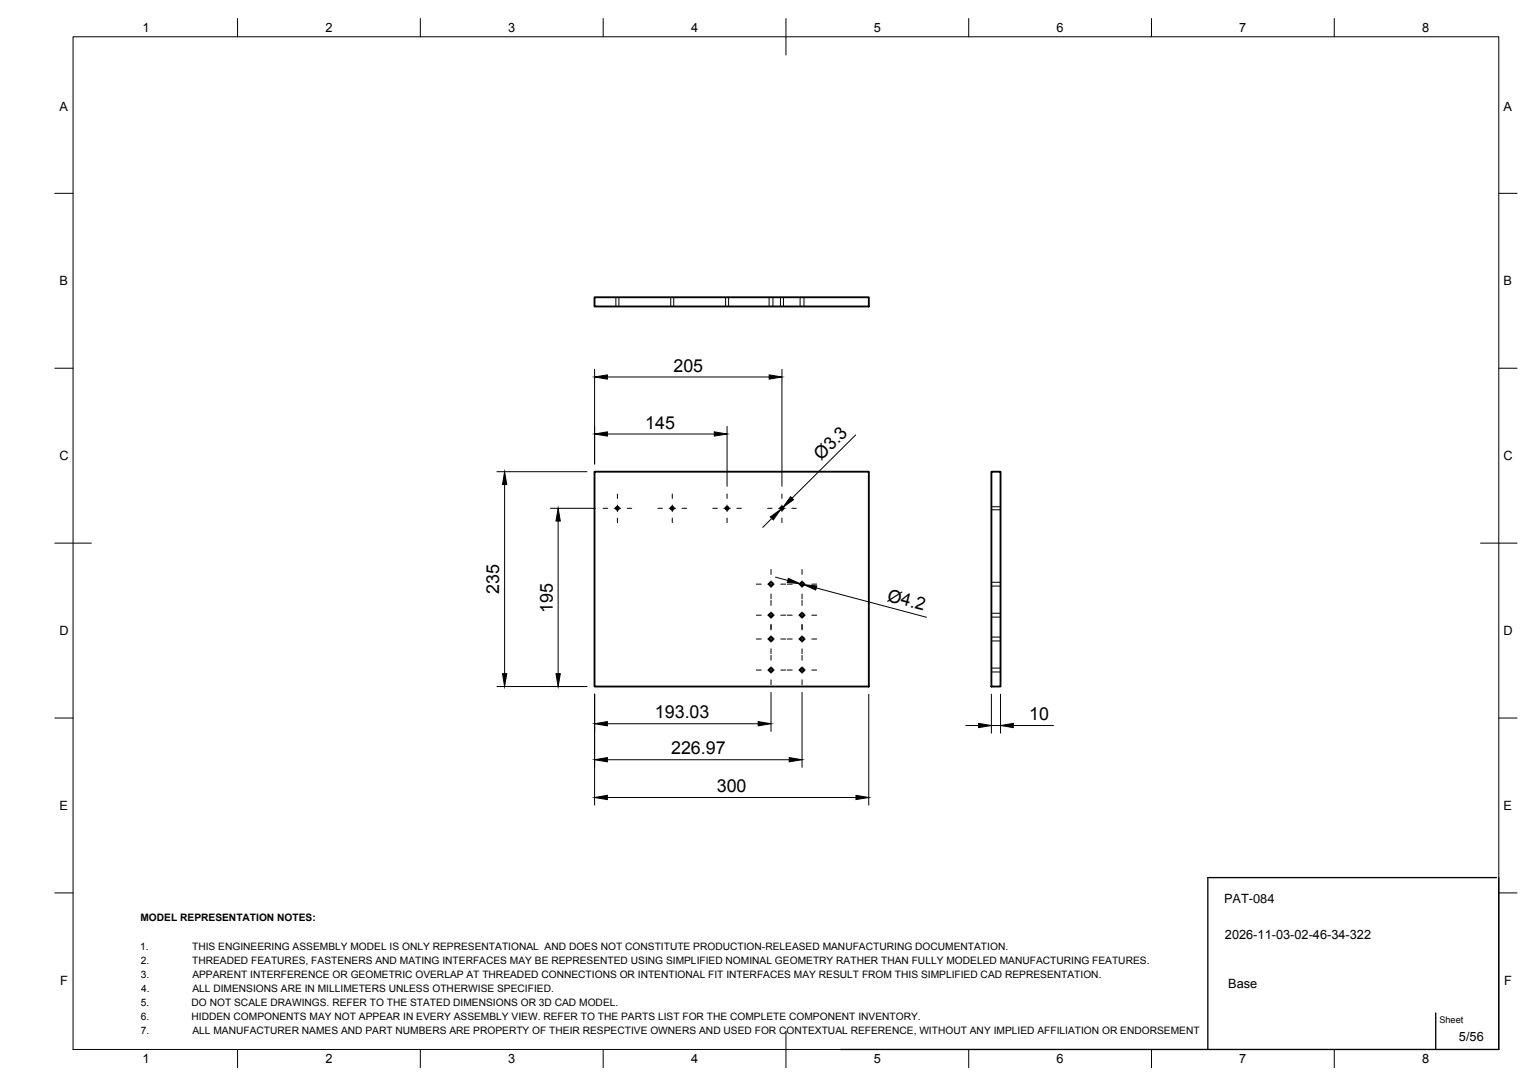
ISO-10303-21;
HEADER;
/* Generated by software containing ST-Developer
 * from STEP Tools, Inc. (www.steptools.com) 
 */

FILE_DESCRIPTION(
/* description */ ('Quick-return (Whitworth) mechanism'),
/* implementation_level */ '2;1');

FILE_NAME(
/* name */ 'Base.step',
/* time_stamp */ '2026-10-28T03:25:57-07:00',
/* author */ (''),
/* organization */ (''),
/* preprocessor_version */ 'ST-DEVELOPER v20.2',
/* originating_system */ 'Autodesk Translation Framework v15.17.0.0',
/* authorisation */ '');

FILE_SCHEMA (('AUTOMOTIVE_DESIGN { 1 0 10303 214 3 1 1 }'));
ENDSEC;

DATA;
#10=MECHANICAL_DESIGN_GEOMETRIC_PRESENTATION_REPRESENTATION('',(#490),#14878);
#402=SHAPE_REPRESENTATION_RELATIONSHIP('SRR','None',#15070,#446);
#446=ADVANCED_BREP_SHAPE_REPRESENTATION('',(#542),#14827);
#490=STYLED_ITEM('',(#15385),#542);
#542=MANIFOLD_SOLID_BREP('Body1',#7844);
#591=FACE_BOUND('',#1530,.T.);
#592=FACE_BOUND('',#1531,.T.);
#593=FACE_BOUND('',#1532,.T.);
#594=FACE_BOUND('',#1533,.T.);
#595=FACE_BOUND('',#1534,.T.);
#596=FACE_BOUND('',#1535,.T.);
#597=FACE_BOUND('',#1536,.T.);
#598=FACE_BOUND('',#1537,.T.);
#599=FACE_BOUND('',#1538,.T.);
#600=FACE_BOUND('',#1539,.T.);
#601=FACE_BOUND('',#1540,.T.);
#602=FACE_BOUND('',#1541,.T.);
#603=FACE_BOUND('',#1543,.T.);
#604=FACE_BOUND('',#1544,.T.);
#605=FACE_BOUND('',#1545,.T.);
#606=FACE_BOUND('',#1546,.T.);
#607=FACE_BOUND('',#1547,.T.);
#608=FACE_BOUND('',#1548,.T.);
#609=FACE_BOUND('',#1549,.T.);
#610=FACE_BOUND('',#1550,.T.);
#611=FACE_BOUND('',#1551,.T.);
#612=FACE_BOUND('',#1552,.T.);
#613=FACE_BOUND('',#1553,.T.);
#614=FACE_BOUND('',#1554,.T.);
#782=PLANE('',#8423);
#783=PLANE('',#8424);
#784=PLANE('',#8425);
#785=PLANE('',#8426);
#786=PLANE('',#8427);
#787=PLANE('',#8428);
#1047=FACE_OUTER_BOUND('',#1513,.T.);
#1048=FACE_OUTER_BOUND('',#1514,.T.);
#1049=FACE_OUTER_BOUND('',#1515,.T.);
#1050=FACE_OUTER_BOUND('',#1516,.T.);
#1051=FACE_OUTER_BOUND('',#1517,.T.);
#1052=FACE_OUTER_BOUND('',#1518,.T.);
#1053=FACE_OUTER_BOUND('',#1519,.T.);
#1054=FACE_OUTER_BOUND('',#1520,.T.);
#1055=FACE_OUTER_BOUND('',#1521,.T.);
#1056=FACE_OUTER_BOUND('',#1522,.T.);
#1057=FACE_OUTER_BOUND('',#1523,.T.);
#1058=FACE_OUTER_BOUND('',#1524,.T.);
#1059=FACE_OUTER_BOUND('',#1525,.T.);
#1060=FACE_OUTER_BOUND('',#1526,.T.);
#1061=FACE_OUTER_BOUND('',#1527,.T.);
#1062=FACE_OUTER_BOUND('',#1528,.T.);
#1063=FACE_OUTER_BOUND('',#1529,.T.);
#1064=FACE_OUTER_BOUND('',#1542,.T.);
#1513=EDGE_LOOP('',(#5262,#5263,#5264,#5265));
#1514=EDGE_LOOP('',(#5266,#5267,#5268,#5269));
#1515=EDGE_LOOP('',(#5270,#5271,#5272,#5273));
#1516=EDGE_LOOP('',(#5274,#5275,#5276,#5277));
#1517=EDGE_LOOP('',(#5278,#5279,#5280,#5281));
#1518=EDGE_LOOP('',(#5282,#5283,#5284,#5285));
#1519=EDGE_LOOP('',(#5286,#5287,#5288,#5289));
#1520=EDGE_LOOP('',(#5290,#5291,#5292,#5293));
#1521=EDGE_LOOP('',(#5294,#5295,#5296,#5297));
#1522=EDGE_LOOP('',(#5298,#5299,#5300,#5301));
#1523=EDGE_LOOP('',(#5302,#5303,#5304,#5305));
#1524=EDGE_LOOP('',(#5306,#5307,#5308,#5309));
#1525=EDGE_LOOP('',(#5310,#5311,#5312,#5313));
#1526=EDGE_LOOP('',(#5314,#5315,#5316,#5317));
#1527=EDGE_LOOP('',(#5318,#5319,#5320,#5321));
#1528=EDGE_LOOP('',(#5322,#5323,#5324,#5325));
#1529=EDGE_LOOP('',(#5326,#5327,#5328,#5329));
#1530=EDGE_LOOP('',(#5330));
#1531=EDGE_LOOP('',(#5331));
#1532=EDGE_LOOP('',(#5332));
#1533=EDGE_LOOP('',(#5333));
#1534=EDGE_LOOP('',(#5334));
#1535=EDGE_LOOP('',(#5335));
#1536=EDGE_LOOP('',(#5336));
#1537=EDGE_LOOP('',(#5337));
#1538=EDGE_LOOP('',(#5338));
#1539=EDGE_LOOP('',(#5339));
#1540=EDGE_LOOP('',(#5340));
#1541=EDGE_LOOP('',(#5341));
#1542=EDGE_LOOP('',(#5342,#5343,#5344,#5345));
#1543=EDGE_LOOP('',(#5346));
#1544=EDGE_LOOP('',(#5347));
#1545=EDGE_LOOP('',(#5348));
#1546=EDGE_LOOP('',(#5349));
#1547=EDGE_LOOP('',(#5350));
#1548=EDGE_LOOP('',(#5351));
#1549=EDGE_LOOP('',(#5352));
#1550=EDGE_LOOP('',(#5353));
#1551=EDGE_LOOP('',(#5354));
#1552=EDGE_LOOP('',(#5355));
#1553=EDGE_LOOP('',(#5356));
#1554=EDGE_LOOP('',(#5357));
#2170=LINE('',#11953,#2693);
#2171=LINE('',#11959,#2694);
#2172=LINE('',#11965,#2695);
#2173=LINE('',#11971,#2696);
#2174=LINE('',#11977,#2697);
#2175=LINE('',#11983,#2698);
#2176=LINE('',#11989,#2699);
#2177=LINE('',#11995,#2700);
#2178=LINE('',#12001,#2701);
#2179=LINE('',#12007,#2702);
#2180=LINE('',#12013,#2703);
#2181=LINE('',#12019,#2704);
#2182=LINE('',#12024,#2705);
#2183=LINE('',#12026,#2706);
#2184=LINE('',#12028,#2707);
#2185=LINE('',#12029,#2708);
#2186=LINE('',#12032,#2709);
#2187=LINE('',#12034,#2710);
#2188=LINE('',#12035,#2711);
#2189=LINE('',#12038,#2712);
#2190=LINE('',#12040,#2713);
#2191=LINE('',#12041,#2714);
#2192=LINE('',#12043,#2715);
#2193=LINE('',#12044,#2716);
#2693=VECTOR('',#9407,0.21);
#2694=VECTOR('',#9414,0.21);
#2695=VECTOR('',#9421,0.21);
#2696=VECTOR('',#9428,0.21);
#2697=VECTOR('',#9435,0.21);
#2698=VECTOR('',#9442,0.21);
#2699=VECTOR('',#9449,0.21);
#2700=VECTOR('',#9456,0.21);
#2701=VECTOR('',#9463,0.164999999999999);
#2702=VECTOR('',#9470,0.164999999999999);
#2703=VECTOR('',#9477,0.165);
#2704=VECTOR('',#9484,0.165);
#2705=VECTOR('',#9489,1.);
#2706=VECTOR('',#9490,1.);
#2707=VECTOR('',#9491,1.);
#2708=VECTOR('',#9492,1.);
#2709=VECTOR('',#9495,1.);
#2710=VECTOR('',#9496,1.);
#2711=VECTOR('',#9497,1.);
#2712=VECTOR('',#9500,1.);
#2713=VECTOR('',#9501,1.);
#2714=VECTOR('',#9502,1.);
#2715=VECTOR('',#9505,1.);
#2716=VECTOR('',#9506,1.);
#3216=CIRCLE('',#8388,0.21);
#3217=CIRCLE('',#8389,0.21);
#3218=CIRCLE('',#8391,0.21);
#3219=CIRCLE('',#8392,0.21);
#3220=CIRCLE('',#8394,0.21);
#3221=CIRCLE('',#8395,0.21);
#3222=CIRCLE('',#8397,0.21);
#3223=CIRCLE('',#8398,0.21);
#3224=CIRCLE('',#8400,0.21);
#3225=CIRCLE('',#8401,0.21);
#3226=CIRCLE('',#8403,0.21);
#3227=CIRCLE('',#8404,0.21);
#3228=CIRCLE('',#8406,0.21);
#3229=CIRCLE('',#8407,0.21);
#3230=CIRCLE('',#8409,0.21);
#3231=CIRCLE('',#8410,0.21);
#3232=CIRCLE('',#8412,0.164999999999999);
#3233=CIRCLE('',#8413,0.164999999999999);
#3234=CIRCLE('',#8415,0.164999999999999);
#3235=CIRCLE('',#8416,0.164999999999999);
#3236=CIRCLE('',#8418,0.165);
#3237=CIRCLE('',#8419,0.165);
#3238=CIRCLE('',#8421,0.165);
#3239=CIRCLE('',#8422,0.165);
#3631=VERTEX_POINT('',#11950);
#3632=VERTEX_POINT('',#11952);
#3633=VERTEX_POINT('',#11956);
#3634=VERTEX_POINT('',#11958);
#3635=VERTEX_POINT('',#11962);
#3636=VERTEX_POINT('',#11964);
#3637=VERTEX_POINT('',#11968);
#3638=VERTEX_POINT('',#11970);
#3639=VERTEX_POINT('',#11974);
#3640=VERTEX_POINT('',#11976);
#3641=VERTEX_POINT('',#11980);
#3642=VERTEX_POINT('',#11982);
#3643=VERTEX_POINT('',#11986);
#3644=VERTEX_POINT('',#11988);
#3645=VERTEX_POINT('',#11992);
#3646=VERTEX_POINT('',#11994);
#3647=VERTEX_POINT('',#11998);
#3648=VERTEX_POINT('',#12000);
#3649=VERTEX_POINT('',#12004);
#3650=VERTEX_POINT('',#12006);
#3651=VERTEX_POINT('',#12010);
#3652=VERTEX_POINT('',#12012);
#3653=VERTEX_POINT('',#12016);
#3654=VERTEX_POINT('',#12018);
#3655=VERTEX_POINT('',#12022);
#3656=VERTEX_POINT('',#12023);
#3657=VERTEX_POINT('',#12025);
#3658=VERTEX_POINT('',#12027);
#3659=VERTEX_POINT('',#12031);
#3660=VERTEX_POINT('',#12033);
#3661=VERTEX_POINT('',#12037);
#3662=VERTEX_POINT('',#12039);
#4288=EDGE_CURVE('',#3631,#3631,#3216,.T.);
#4289=EDGE_CURVE('',#3631,#3632,#2170,.T.);
#4290=EDGE_CURVE('',#3632,#3632,#3217,.T.);
#4291=EDGE_CURVE('',#3633,#3633,#3218,.T.);
#4292=EDGE_CURVE('',#3633,#3634,#2171,.T.);
#4293=EDGE_CURVE('',#3634,#3634,#3219,.T.);
#4294=EDGE_CURVE('',#3635,#3635,#3220,.T.);
#4295=EDGE_CURVE('',#3635,#3636,#2172,.T.);
#4296=EDGE_CURVE('',#3636,#3636,#3221,.T.);
#4297=EDGE_CURVE('',#3637,#3637,#3222,.T.);
#4298=EDGE_CURVE('',#3637,#3638,#2173,.T.);
#4299=EDGE_CURVE('',#3638,#3638,#3223,.T.);
#4300=EDGE_CURVE('',#3639,#3639,#3224,.T.);
#4301=EDGE_CURVE('',#3639,#3640,#2174,.T.);
#4302=EDGE_CURVE('',#3640,#3640,#3225,.T.);
#4303=EDGE_CURVE('',#3641,#3641,#3226,.T.);
#4304=EDGE_CURVE('',#3641,#3642,#2175,.T.);
#4305=EDGE_CURVE('',#3642,#3642,#3227,.T.);
#4306=EDGE_CURVE('',#3643,#3643,#3228,.T.);
#4307=EDGE_CURVE('',#3643,#3644,#2176,.T.);
#4308=EDGE_CURVE('',#3644,#3644,#3229,.T.);
#4309=EDGE_CURVE('',#3645,#3645,#3230,.T.);
#4310=EDGE_CURVE('',#3645,#3646,#2177,.T.);
#4311=EDGE_CURVE('',#3646,#3646,#3231,.T.);
#4312=EDGE_CURVE('',#3647,#3647,#3232,.T.);
#4313=EDGE_CURVE('',#3647,#3648,#2178,.T.);
#4314=EDGE_CURVE('',#3648,#3648,#3233,.T.);
#4315=EDGE_CURVE('',#3649,#3649,#3234,.T.);
#4316=EDGE_CURVE('',#3649,#3650,#2179,.T.);
#4317=EDGE_CURVE('',#3650,#3650,#3235,.T.);
#4318=EDGE_CURVE('',#3651,#3651,#3236,.T.);
#4319=EDGE_CURVE('',#3651,#3652,#2180,.T.);
#4320=EDGE_CURVE('',#3652,#3652,#3237,.T.);
#4321=EDGE_CURVE('',#3653,#3653,#3238,.T.);
#4322=EDGE_CURVE('',#3653,#3654,#2181,.T.);
#4323=EDGE_CURVE('',#3654,#3654,#3239,.T.);
#4324=EDGE_CURVE('',#3655,#3656,#2182,.T.);
#4325=EDGE_CURVE('',#3656,#3657,#2183,.T.);
#4326=EDGE_CURVE('',#3658,#3657,#2184,.T.);
#4327=EDGE_CURVE('',#3655,#3658,#2185,.T.);
#4328=EDGE_CURVE('',#3659,#3655,#2186,.T.);
#4329=EDGE_CURVE('',#3660,#3658,#2187,.T.);
#4330=EDGE_CURVE('',#3659,#3660,#2188,.T.);
#4331=EDGE_CURVE('',#3661,#3659,#2189,.T.);
#4332=EDGE_CURVE('',#3662,#3660,#2190,.T.);
#4333=EDGE_CURVE('',#3661,#3662,#2191,.T.);
#4334=EDGE_CURVE('',#3656,#3661,#2192,.T.);
#4335=EDGE_CURVE('',#3657,#3662,#2193,.T.);
#5262=ORIENTED_EDGE('',*,*,#4288,.F.);
#5263=ORIENTED_EDGE('',*,*,#4289,.T.);
#5264=ORIENTED_EDGE('',*,*,#4290,.F.);
#5265=ORIENTED_EDGE('',*,*,#4289,.F.);
#5266=ORIENTED_EDGE('',*,*,#4291,.F.);
#5267=ORIENTED_EDGE('',*,*,#4292,.T.);
#5268=ORIENTED_EDGE('',*,*,#4293,.F.);
#5269=ORIENTED_EDGE('',*,*,#4292,.F.);
#5270=ORIENTED_EDGE('',*,*,#4294,.F.);
#5271=ORIENTED_EDGE('',*,*,#4295,.T.);
#5272=ORIENTED_EDGE('',*,*,#4296,.F.);
#5273=ORIENTED_EDGE('',*,*,#4295,.F.);
#5274=ORIENTED_EDGE('',*,*,#4297,.F.);
#5275=ORIENTED_EDGE('',*,*,#4298,.T.);
#5276=ORIENTED_EDGE('',*,*,#4299,.F.);
#5277=ORIENTED_EDGE('',*,*,#4298,.F.);
#5278=ORIENTED_EDGE('',*,*,#4300,.F.);
#5279=ORIENTED_EDGE('',*,*,#4301,.T.);
#5280=ORIENTED_EDGE('',*,*,#4302,.F.);
#5281=ORIENTED_EDGE('',*,*,#4301,.F.);
#5282=ORIENTED_EDGE('',*,*,#4303,.F.);
#5283=ORIENTED_EDGE('',*,*,#4304,.T.);
#5284=ORIENTED_EDGE('',*,*,#4305,.F.);
#5285=ORIENTED_EDGE('',*,*,#4304,.F.);
#5286=ORIENTED_EDGE('',*,*,#4306,.F.);
#5287=ORIENTED_EDGE('',*,*,#4307,.T.);
#5288=ORIENTED_EDGE('',*,*,#4308,.F.);
#5289=ORIENTED_EDGE('',*,*,#4307,.F.);
#5290=ORIENTED_EDGE('',*,*,#4309,.F.);
#5291=ORIENTED_EDGE('',*,*,#4310,.T.);
#5292=ORIENTED_EDGE('',*,*,#4311,.F.);
#5293=ORIENTED_EDGE('',*,*,#4310,.F.);
#5294=ORIENTED_EDGE('',*,*,#4312,.F.);
#5295=ORIENTED_EDGE('',*,*,#4313,.T.);
#5296=ORIENTED_EDGE('',*,*,#4314,.F.);
#5297=ORIENTED_EDGE('',*,*,#4313,.F.);
#5298=ORIENTED_EDGE('',*,*,#4315,.F.);
#5299=ORIENTED_EDGE('',*,*,#4316,.T.);
#5300=ORIENTED_EDGE('',*,*,#4317,.F.);
#5301=ORIENTED_EDGE('',*,*,#4316,.F.);
#5302=ORIENTED_EDGE('',*,*,#4318,.F.);
#5303=ORIENTED_EDGE('',*,*,#4319,.T.);
#5304=ORIENTED_EDGE('',*,*,#4320,.F.);
#5305=ORIENTED_EDGE('',*,*,#4319,.F.);
#5306=ORIENTED_EDGE('',*,*,#4321,.F.);
#5307=ORIENTED_EDGE('',*,*,#4322,.T.);
#5308=ORIENTED_EDGE('',*,*,#4323,.F.);
#5309=ORIENTED_EDGE('',*,*,#4322,.F.);
#5310=ORIENTED_EDGE('',*,*,#4324,.T.);
#5311=ORIENTED_EDGE('',*,*,#4325,.T.);
#5312=ORIENTED_EDGE('',*,*,#4326,.F.);
#5313=ORIENTED_EDGE('',*,*,#4327,.F.);
#5314=ORIENTED_EDGE('',*,*,#4328,.T.);
#5315=ORIENTED_EDGE('',*,*,#4327,.T.);
#5316=ORIENTED_EDGE('',*,*,#4329,.F.);
#5317=ORIENTED_EDGE('',*,*,#4330,.F.);
#5318=ORIENTED_EDGE('',*,*,#4331,.T.);
#5319=ORIENTED_EDGE('',*,*,#4330,.T.);
#5320=ORIENTED_EDGE('',*,*,#4332,.F.);
#5321=ORIENTED_EDGE('',*,*,#4333,.F.);
#5322=ORIENTED_EDGE('',*,*,#4334,.T.);
#5323=ORIENTED_EDGE('',*,*,#4333,.T.);
#5324=ORIENTED_EDGE('',*,*,#4335,.F.);
#5325=ORIENTED_EDGE('',*,*,#4325,.F.);
#5326=ORIENTED_EDGE('',*,*,#4335,.T.);
#5327=ORIENTED_EDGE('',*,*,#4332,.T.);
#5328=ORIENTED_EDGE('',*,*,#4329,.T.);
#5329=ORIENTED_EDGE('',*,*,#4326,.T.);
#5330=ORIENTED_EDGE('',*,*,#4302,.T.);
#5331=ORIENTED_EDGE('',*,*,#4305,.T.);
#5332=ORIENTED_EDGE('',*,*,#4308,.T.);
#5333=ORIENTED_EDGE('',*,*,#4311,.T.);
#5334=ORIENTED_EDGE('',*,*,#4314,.T.);
#5335=ORIENTED_EDGE('',*,*,#4317,.T.);
#5336=ORIENTED_EDGE('',*,*,#4320,.T.);
#5337=ORIENTED_EDGE('',*,*,#4323,.T.);
#5338=ORIENTED_EDGE('',*,*,#4299,.T.);
#5339=ORIENTED_EDGE('',*,*,#4296,.T.);
#5340=ORIENTED_EDGE('',*,*,#4293,.T.);
#5341=ORIENTED_EDGE('',*,*,#4290,.T.);
#5342=ORIENTED_EDGE('',*,*,#4334,.F.);
#5343=ORIENTED_EDGE('',*,*,#4324,.F.);
#5344=ORIENTED_EDGE('',*,*,#4328,.F.);
#5345=ORIENTED_EDGE('',*,*,#4331,.F.);
#5346=ORIENTED_EDGE('',*,*,#4300,.T.);
#5347=ORIENTED_EDGE('',*,*,#4303,.T.);
#5348=ORIENTED_EDGE('',*,*,#4306,.T.);
#5349=ORIENTED_EDGE('',*,*,#4309,.T.);
#5350=ORIENTED_EDGE('',*,*,#4312,.T.);
#5351=ORIENTED_EDGE('',*,*,#4315,.T.);
#5352=ORIENTED_EDGE('',*,*,#4318,.T.);
#5353=ORIENTED_EDGE('',*,*,#4321,.T.);
#5354=ORIENTED_EDGE('',*,*,#4297,.T.);
#5355=ORIENTED_EDGE('',*,*,#4294,.T.);
#5356=ORIENTED_EDGE('',*,*,#4291,.T.);
#5357=ORIENTED_EDGE('',*,*,#4288,.T.);
#7210=CYLINDRICAL_SURFACE('',#8387,0.21);
#7211=CYLINDRICAL_SURFACE('',#8390,0.21);
#7212=CYLINDRICAL_SURFACE('',#8393,0.21);
#7213=CYLINDRICAL_SURFACE('',#8396,0.21);
#7214=CYLINDRICAL_SURFACE('',#8399,0.21);
#7215=CYLINDRICAL_SURFACE('',#8402,0.21);
#7216=CYLINDRICAL_SURFACE('',#8405,0.21);
#7217=CYLINDRICAL_SURFACE('',#8408,0.21);
#7218=CYLINDRICAL_SURFACE('',#8411,0.164999999999999);
#7219=CYLINDRICAL_SURFACE('',#8414,0.164999999999999);
#7220=CYLINDRICAL_SURFACE('',#8417,0.165);
#7221=CYLINDRICAL_SURFACE('',#8420,0.165);
#7378=ADVANCED_FACE('',(#1047),#7210,.F.);
#7379=ADVANCED_FACE('',(#1048),#7211,.F.);
#7380=ADVANCED_FACE('',(#1049),#7212,.F.);
#7381=ADVANCED_FACE('',(#1050),#7213,.F.);
#7382=ADVANCED_FACE('',(#1051),#7214,.F.);
#7383=ADVANCED_FACE('',(#1052),#7215,.F.);
#7384=ADVANCED_FACE('',(#1053),#7216,.F.);
#7385=ADVANCED_FACE('',(#1054),#7217,.F.);
#7386=ADVANCED_FACE('',(#1055),#7218,.F.);
#7387=ADVANCED_FACE('',(#1056),#7219,.F.);
#7388=ADVANCED_FACE('',(#1057),#7220,.F.);
#7389=ADVANCED_FACE('',(#1058),#7221,.F.);
#7390=ADVANCED_FACE('',(#1059),#782,.T.);
#7391=ADVANCED_FACE('',(#1060),#783,.T.);
#7392=ADVANCED_FACE('',(#1061),#784,.T.);
#7393=ADVANCED_FACE('',(#1062),#785,.T.);
#7394=ADVANCED_FACE('',(#1063,#591,#592,#593,#594,#595,#596,#597,#598,#599,
#600,#601,#602),#786,.T.);
#7395=ADVANCED_FACE('',(#1064,#603,#604,#605,#606,#607,#608,#609,#610,#611,
#612,#613,#614),#787,.F.);
#7844=CLOSED_SHELL('',(#7378,#7379,#7380,#7381,#7382,#7383,#7384,#7385,
#7386,#7387,#7388,#7389,#7390,#7391,#7392,#7393,#7394,#7395));
#8386=AXIS2_PLACEMENT_3D('',#11948,#9401,#9402);
#8387=AXIS2_PLACEMENT_3D('',#11949,#9403,#9404);
#8388=AXIS2_PLACEMENT_3D('',#11951,#9405,#9406);
#8389=AXIS2_PLACEMENT_3D('',#11954,#9408,#9409);
#8390=AXIS2_PLACEMENT_3D('',#11955,#9410,#9411);
#8391=AXIS2_PLACEMENT_3D('',#11957,#9412,#9413);
#8392=AXIS2_PLACEMENT_3D('',#11960,#9415,#9416);
#8393=AXIS2_PLACEMENT_3D('',#11961,#9417,#9418);
#8394=AXIS2_PLACEMENT_3D('',#11963,#9419,#9420);
#8395=AXIS2_PLACEMENT_3D('',#11966,#9422,#9423);
#8396=AXIS2_PLACEMENT_3D('',#11967,#9424,#9425);
#8397=AXIS2_PLACEMENT_3D('',#11969,#9426,#9427);
#8398=AXIS2_PLACEMENT_3D('',#11972,#9429,#9430);
#8399=AXIS2_PLACEMENT_3D('',#11973,#9431,#9432);
#8400=AXIS2_PLACEMENT_3D('',#11975,#9433,#9434);
#8401=AXIS2_PLACEMENT_3D('',#11978,#9436,#9437);
#8402=AXIS2_PLACEMENT_3D('',#11979,#9438,#9439);
#8403=AXIS2_PLACEMENT_3D('',#11981,#9440,#9441);
#8404=AXIS2_PLACEMENT_3D('',#11984,#9443,#9444);
#8405=AXIS2_PLACEMENT_3D('',#11985,#9445,#9446);
#8406=AXIS2_PLACEMENT_3D('',#11987,#9447,#9448);
#8407=AXIS2_PLACEMENT_3D('',#11990,#9450,#9451);
#8408=AXIS2_PLACEMENT_3D('',#11991,#9452,#9453);
#8409=AXIS2_PLACEMENT_3D('',#11993,#9454,#9455);
#8410=AXIS2_PLACEMENT_3D('',#11996,#9457,#9458);
#8411=AXIS2_PLACEMENT_3D('',#11997,#9459,#9460);
#8412=AXIS2_PLACEMENT_3D('',#11999,#9461,#9462);
#8413=AXIS2_PLACEMENT_3D('',#12002,#9464,#9465);
#8414=AXIS2_PLACEMENT_3D('',#12003,#9466,#9467);
#8415=AXIS2_PLACEMENT_3D('',#12005,#9468,#9469);
#8416=AXIS2_PLACEMENT_3D('',#12008,#9471,#9472);
#8417=AXIS2_PLACEMENT_3D('',#12009,#9473,#9474);
#8418=AXIS2_PLACEMENT_3D('',#12011,#9475,#9476);
#8419=AXIS2_PLACEMENT_3D('',#12014,#9478,#9479);
#8420=AXIS2_PLACEMENT_3D('',#12015,#9480,#9481);
#8421=AXIS2_PLACEMENT_3D('',#12017,#9482,#9483);
#8422=AXIS2_PLACEMENT_3D('',#12020,#9485,#9486);
#8423=AXIS2_PLACEMENT_3D('',#12021,#9487,#9488);
#8424=AXIS2_PLACEMENT_3D('',#12030,#9493,#9494);
#8425=AXIS2_PLACEMENT_3D('',#12036,#9498,#9499);
#8426=AXIS2_PLACEMENT_3D('',#12042,#9503,#9504);
#8427=AXIS2_PLACEMENT_3D('',#12045,#9507,#9508);
#8428=AXIS2_PLACEMENT_3D('',#12046,#9509,#9510);
#9401=DIRECTION('axis',(0.,0.,1.));
#9402=DIRECTION('refdir',(1.,0.,0.));
#9403=DIRECTION('center_axis',(0.,0.,1.));
#9404=DIRECTION('ref_axis',(1.,0.,0.));
#9405=DIRECTION('center_axis',(0.,0.,1.));
#9406=DIRECTION('ref_axis',(1.,0.,0.));
#9407=DIRECTION('',(0.,0.,1.));
#9408=DIRECTION('center_axis',(0.,0.,-1.));
#9409=DIRECTION('ref_axis',(1.,0.,0.));
#9410=DIRECTION('center_axis',(0.,0.,1.));
#9411=DIRECTION('ref_axis',(1.,0.,0.));
#9412=DIRECTION('center_axis',(0.,0.,1.));
#9413=DIRECTION('ref_axis',(1.,0.,0.));
#9414=DIRECTION('',(0.,0.,1.));
#9415=DIRECTION('center_axis',(0.,0.,-1.));
#9416=DIRECTION('ref_axis',(1.,0.,0.));
#9417=DIRECTION('center_axis',(0.,0.,1.));
#9418=DIRECTION('ref_axis',(1.,0.,0.));
#9419=DIRECTION('center_axis',(0.,0.,1.));
#9420=DIRECTION('ref_axis',(1.,0.,0.));
#9421=DIRECTION('',(0.,0.,1.));
#9422=DIRECTION('center_axis',(0.,0.,-1.));
#9423=DIRECTION('ref_axis',(1.,0.,0.));
#9424=DIRECTION('center_axis',(0.,0.,1.));
#9425=DIRECTION('ref_axis',(1.,0.,0.));
#9426=DIRECTION('center_axis',(0.,0.,1.));
#9427=DIRECTION('ref_axis',(1.,0.,0.));
#9428=DIRECTION('',(0.,0.,1.));
#9429=DIRECTION('center_axis',(0.,0.,-1.));
#9430=DIRECTION('ref_axis',(1.,0.,0.));
#9431=DIRECTION('center_axis',(0.,0.,1.));
#9432=DIRECTION('ref_axis',(1.,0.,0.));
#9433=DIRECTION('center_axis',(0.,0.,1.));
#9434=DIRECTION('ref_axis',(1.,0.,0.));
#9435=DIRECTION('',(0.,0.,1.));
#9436=DIRECTION('center_axis',(0.,0.,-1.));
#9437=DIRECTION('ref_axis',(1.,0.,0.));
#9438=DIRECTION('center_axis',(0.,0.,1.));
#9439=DIRECTION('ref_axis',(1.,0.,0.));
#9440=DIRECTION('center_axis',(0.,0.,1.));
#9441=DIRECTION('ref_axis',(1.,0.,0.));
#9442=DIRECTION('',(0.,0.,1.));
#9443=DIRECTION('center_axis',(0.,0.,-1.));
#9444=DIRECTION('ref_axis',(1.,0.,0.));
#9445=DIRECTION('center_axis',(0.,0.,1.));
#9446=DIRECTION('ref_axis',(1.,0.,0.));
#9447=DIRECTION('center_axis',(0.,0.,1.));
#9448=DIRECTION('ref_axis',(1.,0.,0.));
#9449=DIRECTION('',(0.,0.,1.));
#9450=DIRECTION('center_axis',(0.,0.,-1.));
#9451=DIRECTION('ref_axis',(1.,0.,0.));
#9452=DIRECTION('center_axis',(0.,0.,1.));
#9453=DIRECTION('ref_axis',(1.,0.,0.));
#9454=DIRECTION('center_axis',(0.,0.,1.));
#9455=DIRECTION('ref_axis',(1.,0.,0.));
#9456=DIRECTION('',(0.,0.,1.));
#9457=DIRECTION('center_axis',(0.,0.,-1.));
#9458=DIRECTION('ref_axis',(1.,0.,0.));
#9459=DIRECTION('center_axis',(0.,0.,1.));
#9460=DIRECTION('ref_axis',(1.,0.,0.));
#9461=DIRECTION('center_axis',(0.,0.,1.));
#9462=DIRECTION('ref_axis',(1.,0.,0.));
#9463=DIRECTION('',(0.,0.,1.));
#9464=DIRECTION('center_axis',(0.,0.,-1.));
#9465=DIRECTION('ref_axis',(1.,0.,0.));
#9466=DIRECTION('center_axis',(0.,0.,1.));
#9467=DIRECTION('ref_axis',(1.,0.,0.));
#9468=DIRECTION('center_axis',(0.,0.,1.));
#9469=DIRECTION('ref_axis',(1.,0.,0.));
#9470=DIRECTION('',(0.,0.,1.));
#9471=DIRECTION('center_axis',(0.,0.,-1.));
#9472=DIRECTION('ref_axis',(1.,0.,0.));
#9473=DIRECTION('center_axis',(0.,0.,1.));
#9474=DIRECTION('ref_axis',(1.,0.,0.));
#9475=DIRECTION('center_axis',(0.,0.,1.));
#9476=DIRECTION('ref_axis',(1.,0.,0.));
#9477=DIRECTION('',(0.,0.,1.));
#9478=DIRECTION('center_axis',(0.,0.,-1.));
#9479=DIRECTION('ref_axis',(1.,0.,0.));
#9480=DIRECTION('center_axis',(0.,0.,1.));
#9481=DIRECTION('ref_axis',(1.,0.,0.));
#9482=DIRECTION('center_axis',(0.,0.,1.));
#9483=DIRECTION('ref_axis',(1.,0.,0.));
#9484=DIRECTION('',(0.,0.,1.));
#9485=DIRECTION('center_axis',(0.,0.,-1.));
#9486=DIRECTION('ref_axis',(1.,0.,0.));
#9487=DIRECTION('center_axis',(0.,1.,0.));
#9488=DIRECTION('ref_axis',(-1.,0.,0.));
#9489=DIRECTION('',(-1.,0.,0.));
#9490=DIRECTION('',(0.,0.,1.));
#9491=DIRECTION('',(-1.,0.,0.));
#9492=DIRECTION('',(0.,0.,1.));
#9493=DIRECTION('center_axis',(1.,0.,0.));
#9494=DIRECTION('ref_axis',(0.,1.,0.));
#9495=DIRECTION('',(0.,1.,0.));
#9496=DIRECTION('',(0.,1.,0.));
#9497=DIRECTION('',(0.,0.,1.));
#9498=DIRECTION('center_axis',(0.,-1.,0.));
#9499=DIRECTION('ref_axis',(1.,0.,0.));
#9500=DIRECTION('',(1.,0.,0.));
#9501=DIRECTION('',(1.,0.,0.));
#9502=DIRECTION('',(0.,0.,1.));
#9503=DIRECTION('center_axis',(-1.,0.,0.));
#9504=DIRECTION('ref_axis',(0.,-1.,0.));
#9505=DIRECTION('',(0.,-1.,0.));
#9506=DIRECTION('',(0.,-1.,0.));
#9507=DIRECTION('center_axis',(0.,0.,1.));
#9508=DIRECTION('ref_axis',(1.,0.,0.));
#9509=DIRECTION('center_axis',(0.,0.,1.));
#9510=DIRECTION('ref_axis',(1.,0.,0.));
#11948=CARTESIAN_POINT('',(0.,0.,0.));
#11949=CARTESIAN_POINT('Origin',(-1.69705627484771,4.30294372515229,-0.1));
#11950=CARTESIAN_POINT('',(-1.90705627484771,4.30294372515229,0.));
#11951=CARTESIAN_POINT('Origin',(-1.69705627484771,4.30294372515229,0.));
#11952=CARTESIAN_POINT('',(-1.90705627484771,4.30294372515229,1.));
#11953=CARTESIAN_POINT('',(-1.90705627484771,4.30294372515229,-0.1));
#11954=CARTESIAN_POINT('Origin',(-1.69705627484771,4.30294372515229,1.));
#11955=CARTESIAN_POINT('Origin',(-1.69705627484771,7.69705627484771,-0.1));
#11956=CARTESIAN_POINT('',(-1.90705627484771,7.69705627484771,0.));
#11957=CARTESIAN_POINT('Origin',(-1.69705627484771,7.69705627484771,0.));
#11958=CARTESIAN_POINT('',(-1.90705627484771,7.69705627484771,1.));
#11959=CARTESIAN_POINT('',(-1.90705627484771,7.69705627484771,-0.1));
#11960=CARTESIAN_POINT('Origin',(-1.69705627484771,7.69705627484771,1.));
#11961=CARTESIAN_POINT('Origin',(1.69705627484771,7.69705627484771,-0.1));
#11962=CARTESIAN_POINT('',(1.48705627484771,7.69705627484771,0.));
#11963=CARTESIAN_POINT('Origin',(1.69705627484771,7.69705627484771,0.));
#11964=CARTESIAN_POINT('',(1.48705627484771,7.69705627484771,1.));
#11965=CARTESIAN_POINT('',(1.48705627484771,7.69705627484771,-0.1));
#11966=CARTESIAN_POINT('Origin',(1.69705627484771,7.69705627484771,1.));
#11967=CARTESIAN_POINT('Origin',(1.69705627484771,4.30294372515229,-0.1));
#11968=CARTESIAN_POINT('',(1.48705627484771,4.30294372515229,0.));
#11969=CARTESIAN_POINT('Origin',(1.69705627484771,4.30294372515229,0.));
#11970=CARTESIAN_POINT('',(1.48705627484771,4.30294372515229,1.));
#11971=CARTESIAN_POINT('',(1.48705627484771,4.30294372515229,-0.1));
#11972=CARTESIAN_POINT('Origin',(1.69705627484771,4.30294372515229,1.));
#11973=CARTESIAN_POINT('Origin',(-1.69705627484771,-1.69705627484771,-0.1));
#11974=CARTESIAN_POINT('',(-1.90705627484771,-1.69705627484771,0.));
#11975=CARTESIAN_POINT('Origin',(-1.69705627484771,-1.69705627484771,0.));
#11976=CARTESIAN_POINT('',(-1.90705627484771,-1.69705627484771,1.));
#11977=CARTESIAN_POINT('',(-1.90705627484771,-1.69705627484771,-0.1));
#11978=CARTESIAN_POINT('Origin',(-1.69705627484771,-1.69705627484771,1.));
#11979=CARTESIAN_POINT('Origin',(-1.69705627484771,1.69705627484771,-0.1));
#11980=CARTESIAN_POINT('',(-1.90705627484771,1.69705627484771,0.));
#11981=CARTESIAN_POINT('Origin',(-1.69705627484771,1.69705627484771,0.));
#11982=CARTESIAN_POINT('',(-1.90705627484771,1.69705627484771,1.));
#11983=CARTESIAN_POINT('',(-1.90705627484771,1.69705627484771,-0.1));
#11984=CARTESIAN_POINT('Origin',(-1.69705627484771,1.69705627484771,1.));
#11985=CARTESIAN_POINT('Origin',(1.69705627484771,1.69705627484771,-0.1));
#11986=CARTESIAN_POINT('',(1.48705627484771,1.69705627484771,0.));
#11987=CARTESIAN_POINT('Origin',(1.69705627484771,1.69705627484771,0.));
#11988=CARTESIAN_POINT('',(1.48705627484771,1.69705627484771,1.));
#11989=CARTESIAN_POINT('',(1.48705627484771,1.69705627484771,-0.1));
#11990=CARTESIAN_POINT('Origin',(1.69705627484771,1.69705627484771,1.));
#11991=CARTESIAN_POINT('Origin',(1.69705627484771,-1.69705627484771,-0.1));
#11992=CARTESIAN_POINT('',(1.48705627484771,-1.69705627484771,0.));
#11993=CARTESIAN_POINT('Origin',(1.69705627484771,-1.69705627484771,0.));
#11994=CARTESIAN_POINT('',(1.48705627484771,-1.69705627484771,1.));
#11995=CARTESIAN_POINT('',(1.48705627484771,-1.69705627484771,-0.1));
#11996=CARTESIAN_POINT('Origin',(1.69705627484771,-1.69705627484771,1.));
#11997=CARTESIAN_POINT('Origin',(18.5,16.,-0.1));
#11998=CARTESIAN_POINT('',(18.335,16.,0.));
#11999=CARTESIAN_POINT('Origin',(18.5,16.,0.));
#12000=CARTESIAN_POINT('',(18.335,16.,1.));
#12001=CARTESIAN_POINT('',(18.335,16.,-0.1));
#12002=CARTESIAN_POINT('Origin',(18.5,16.,1.));
#12003=CARTESIAN_POINT('Origin',(12.5,16.,-0.1));
#12004=CARTESIAN_POINT('',(12.335,16.,0.));
#12005=CARTESIAN_POINT('Origin',(12.5,16.,0.));
#12006=CARTESIAN_POINT('',(12.335,16.,1.));
#12007=CARTESIAN_POINT('',(12.335,16.,-0.1));
#12008=CARTESIAN_POINT('Origin',(12.5,16.,1.));
#12009=CARTESIAN_POINT('Origin',(6.5,16.,-0.1));
#12010=CARTESIAN_POINT('',(6.335,16.,0.));
#12011=CARTESIAN_POINT('Origin',(6.5,16.,0.));
#12012=CARTESIAN_POINT('',(6.335,16.,1.));
#12013=CARTESIAN_POINT('',(6.335,16.,-0.1));
#12014=CARTESIAN_POINT('Origin',(6.5,16.,1.));
#12015=CARTESIAN_POINT('Origin',(0.5,16.,-0.1));
#12016=CARTESIAN_POINT('',(0.335,16.,0.));
#12017=CARTESIAN_POINT('Origin',(0.5,16.,0.));
#12018=CARTESIAN_POINT('',(0.335,16.,1.));
#12019=CARTESIAN_POINT('',(0.335,16.,-0.1));
#12020=CARTESIAN_POINT('Origin',(0.5,16.,1.));
#12021=CARTESIAN_POINT('Origin',(21.,20.,0.));
#12022=CARTESIAN_POINT('',(21.,20.,0.));
#12023=CARTESIAN_POINT('',(-9.,20.,0.));
#12024=CARTESIAN_POINT('',(21.,20.,0.));
#12025=CARTESIAN_POINT('',(-9.,20.,1.));
#12026=CARTESIAN_POINT('',(-9.,20.,0.));
#12027=CARTESIAN_POINT('',(21.,20.,1.));
#12028=CARTESIAN_POINT('',(21.,20.,1.));
#12029=CARTESIAN_POINT('',(21.,20.,0.));
#12030=CARTESIAN_POINT('Origin',(21.,-3.5,0.));
#12031=CARTESIAN_POINT('',(21.,-3.5,0.));
#12032=CARTESIAN_POINT('',(21.,-3.5,0.));
#12033=CARTESIAN_POINT('',(21.,-3.5,1.));
#12034=CARTESIAN_POINT('',(21.,-3.5,1.));
#12035=CARTESIAN_POINT('',(21.,-3.5,0.));
#12036=CARTESIAN_POINT('Origin',(-9.,-3.5,0.));
#12037=CARTESIAN_POINT('',(-9.,-3.5,0.));
#12038=CARTESIAN_POINT('',(-9.,-3.5,0.));
#12039=CARTESIAN_POINT('',(-9.,-3.5,1.));
#12040=CARTESIAN_POINT('',(-9.,-3.5,1.));
#12041=CARTESIAN_POINT('',(-9.,-3.5,0.));
#12042=CARTESIAN_POINT('Origin',(-9.,20.,0.));
#12043=CARTESIAN_POINT('',(-9.,20.,0.));
#12044=CARTESIAN_POINT('',(-9.,20.,1.));
#12045=CARTESIAN_POINT('Origin',(6.,8.25,1.));
#12046=CARTESIAN_POINT('Origin',(6.,8.25,0.));
#14773=UNCERTAINTY_MEASURE_WITH_UNIT(LENGTH_MEASURE(0.001),#14879,
'DISTANCE_ACCURACY_VALUE',
'Maximum model space distance between geometric entities at asserted c
onnectivities');
#14824=UNCERTAINTY_MEASURE_WITH_UNIT(LENGTH_MEASURE(0.001),#14879,
'DISTANCE_ACCURACY_VALUE',
'Maximum model space distance between geometric entities at asserted c
onnectivities');
#14827=(
GEOMETRIC_REPRESENTATION_CONTEXT(3)
GLOBAL_UNCERTAINTY_ASSIGNED_CONTEXT((#14773))
GLOBAL_UNIT_ASSIGNED_CONTEXT((#14879,#14881,#14882))
REPRESENTATION_CONTEXT('','3D')
);
#14878=(
GEOMETRIC_REPRESENTATION_CONTEXT(3)
GLOBAL_UNCERTAINTY_ASSIGNED_CONTEXT((#14824))
GLOBAL_UNIT_ASSIGNED_CONTEXT((#14879,#14881,#14882))
REPRESENTATION_CONTEXT('','3D')
);
#14879=(
LENGTH_UNIT()
NAMED_UNIT(*)
SI_UNIT(.CENTI.,.METRE.)
);
#14881=(
NAMED_UNIT(*)
PLANE_ANGLE_UNIT()
SI_UNIT($,.RADIAN.)
);
#14882=(
NAMED_UNIT(*)
SI_UNIT($,.STERADIAN.)
SOLID_ANGLE_UNIT()
);
#14885=SHAPE_DEFINITION_REPRESENTATION(#14938,#15070);
#14938=PRODUCT_DEFINITION_SHAPE('',$,#15124);
#15070=SHAPE_REPRESENTATION('',(#8386),#14827);
#15121=PRODUCT_DEFINITION_CONTEXT('part definition',#15282,'design');
#15124=PRODUCT_DEFINITION('Base','Base',#15177,#15121);
#15177=PRODUCT_DEFINITION_FORMATION('',$,#15286);
#15282=APPLICATION_CONTEXT(
'Core Data for Automotive Mechanical Design Process');
#15283=PRODUCT_CONTEXT('part definition',#15282,'mechanical');
#15286=PRODUCT('Base','Base','Base',(#15283));
#15379=COLOUR_RGB('Dark Blue',0.08,0.2,0.34);
#15380=FILL_AREA_STYLE_COLOUR('',#15379);
#15381=FILL_AREA_STYLE('',(#15380));
#15382=SURFACE_STYLE_FILL_AREA(#15381);
#15383=SURFACE_SIDE_STYLE('',(#15382));
#15384=SURFACE_STYLE_USAGE(.BOTH.,#15383);
#15385=PRESENTATION_STYLE_ASSIGNMENT((#15384));
ENDSEC;
END-ISO-10303-21;
